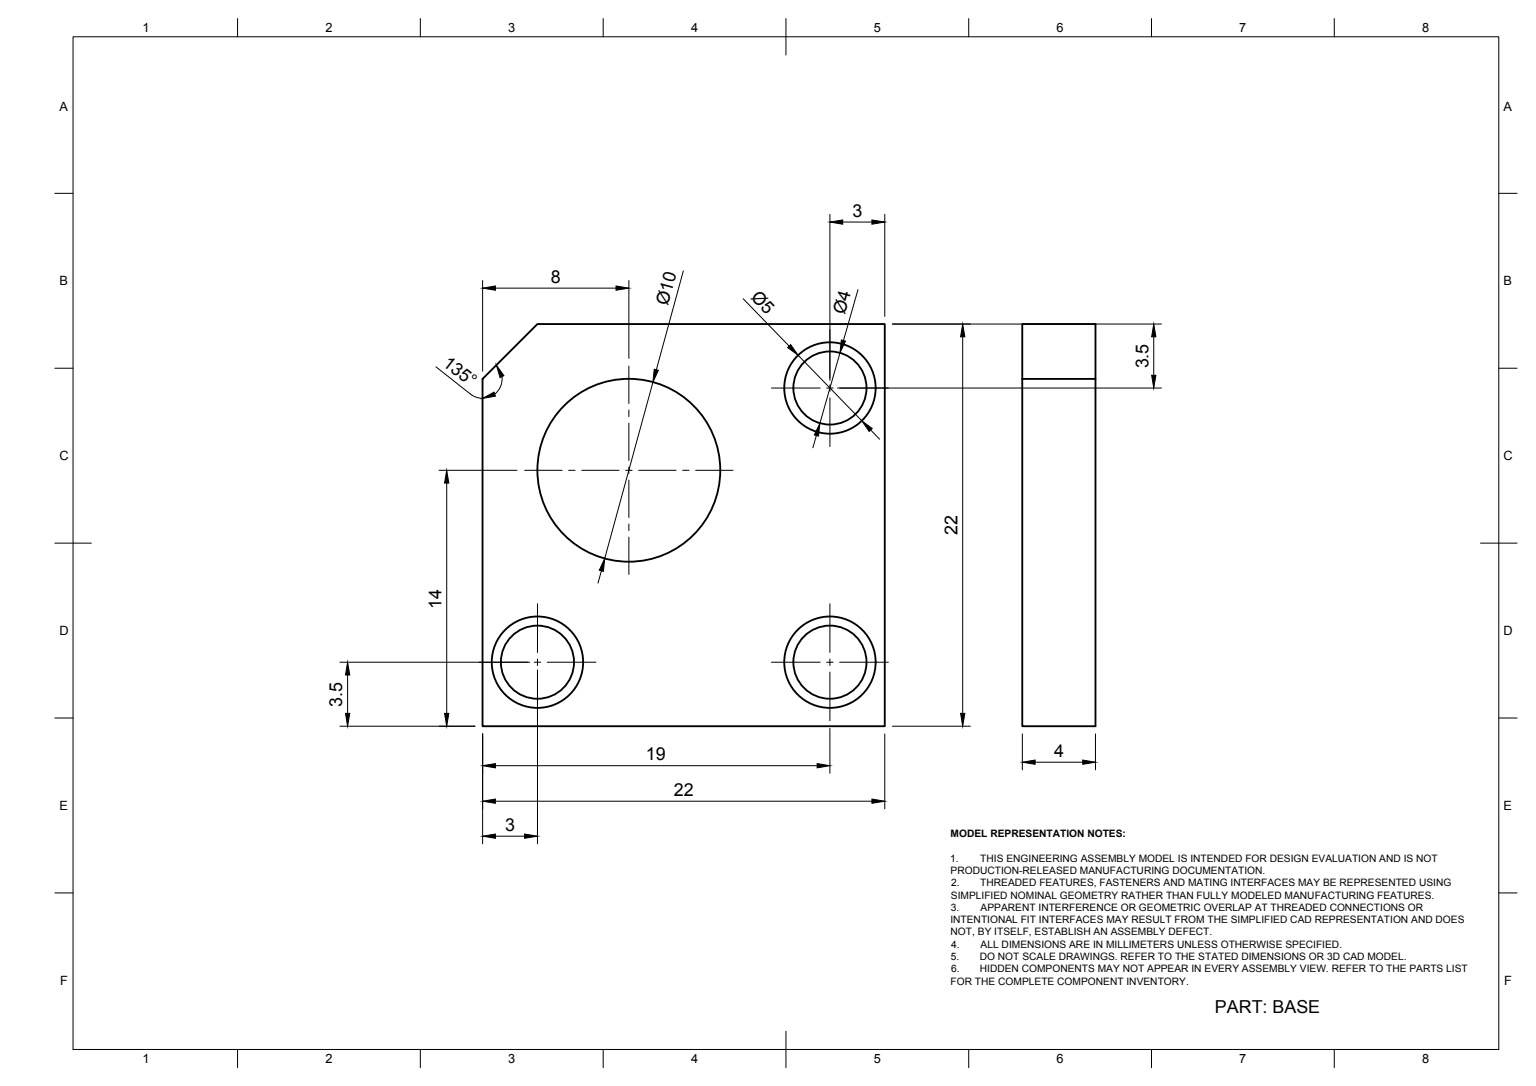
ISO-10303-21;
HEADER;
/* Generated by software containing ST-Developer
 * from STEP Tools, Inc. (www.steptools.com) 
 */

FILE_DESCRIPTION(
/* description */ (''),
/* implementation_level */ '2;1');

FILE_NAME(
/* name */ 'Base.step',
/* time_stamp */ '2026-10-04T23:23:09-07:00',
/* author */ (''),
/* organization */ (''),
/* preprocessor_version */ 'ST-DEVELOPER v20.2',
/* originating_system */ 'Autodesk Translation Framework v15.15.0.0',
/* authorisation */ '');

FILE_SCHEMA (('AUTOMOTIVE_DESIGN { 1 0 10303 214 3 1 1 }'));
ENDSEC;

DATA;
#10=MECHANICAL_DESIGN_GEOMETRIC_PRESENTATION_REPRESENTATION('',(#65),#2676);
#49=SHAPE_REPRESENTATION_RELATIONSHIP('SRR','None',#2708,#57);
#57=ADVANCED_BREP_SHAPE_REPRESENTATION('',(#76),#2668);
#65=STYLED_ITEM('',(#2757),#76);
#76=MANIFOLD_SOLID_BREP('Body1',#1476);
#87=CYLINDRICAL_SURFACE('',#1585,2.);
#88=CYLINDRICAL_SURFACE('',#1589,2.);
#89=CYLINDRICAL_SURFACE('',#1593,2.);
#90=CYLINDRICAL_SURFACE('',#1598,5.);
#109=FACE_BOUND('',#287,.T.);
#110=FACE_BOUND('',#288,.T.);
#111=FACE_BOUND('',#289,.T.);
#112=FACE_BOUND('',#290,.T.);
#113=FACE_BOUND('',#306,.T.);
#135=PLANE('',#1581);
#136=PLANE('',#1595);
#137=PLANE('',#1596);
#138=PLANE('',#1597);
#139=PLANE('',#1600);
#140=PLANE('',#1601);
#141=PLANE('',#1602);
#142=PLANE('',#1603);
#143=PLANE('',#1604);
#144=PLANE('',#1605);
#187=FACE_OUTER_BOUND('',#285,.T.);
#188=FACE_OUTER_BOUND('',#286,.T.);
#189=FACE_OUTER_BOUND('',#291,.T.);
#190=FACE_OUTER_BOUND('',#292,.T.);
#191=FACE_OUTER_BOUND('',#293,.T.);
#192=FACE_OUTER_BOUND('',#294,.T.);
#193=FACE_OUTER_BOUND('',#295,.T.);
#194=FACE_OUTER_BOUND('',#296,.T.);
#195=FACE_OUTER_BOUND('',#297,.T.);
#196=FACE_OUTER_BOUND('',#298,.T.);
#197=FACE_OUTER_BOUND('',#299,.T.);
#198=FACE_OUTER_BOUND('',#300,.T.);
#199=FACE_OUTER_BOUND('',#301,.T.);
#200=FACE_OUTER_BOUND('',#302,.T.);
#201=FACE_OUTER_BOUND('',#303,.T.);
#202=FACE_OUTER_BOUND('',#304,.T.);
#203=FACE_OUTER_BOUND('',#305,.T.);
#285=EDGE_LOOP('',(#998,#999,#1000,#1001));
#286=EDGE_LOOP('',(#1002,#1003,#1004,#1005,#1006));
#287=EDGE_LOOP('',(#1007));
#288=EDGE_LOOP('',(#1008));
#289=EDGE_LOOP('',(#1009));
#290=EDGE_LOOP('',(#1010));
#291=EDGE_LOOP('',(#1011,#1012,#1013,#1014));
#292=EDGE_LOOP('',(#1015,#1016,#1017,#1018));
#293=EDGE_LOOP('',(#1019,#1020,#1021,#1022));
#294=EDGE_LOOP('',(#1023,#1024,#1025,#1026));
#295=EDGE_LOOP('',(#1027,#1028,#1029,#1030));
#296=EDGE_LOOP('',(#1031));
#297=EDGE_LOOP('',(#1032));
#298=EDGE_LOOP('',(#1033));
#299=EDGE_LOOP('',(#1034,#1035,#1036,#1037));
#300=EDGE_LOOP('',(#1038,#1039,#1040,#1041));
#301=EDGE_LOOP('',(#1042,#1043,#1044,#1045));
#302=EDGE_LOOP('',(#1046,#1047,#1048,#1049));
#303=EDGE_LOOP('',(#1050,#1051,#1052,#1053));
#304=EDGE_LOOP('',(#1054,#1055,#1056,#1057));
#305=EDGE_LOOP('',(#1058,#1059,#1060,#1061,#1062));
#306=EDGE_LOOP('',(#1063));
#409=LINE('',#2250,#519);
#410=LINE('',#2255,#520);
#411=LINE('',#2257,#521);
#412=LINE('',#2259,#522);
#413=LINE('',#2261,#523);
#414=LINE('',#2262,#524);
#415=LINE('',#2271,#525);
#416=LINE('',#2276,#526);
#417=LINE('',#2279,#527);
#418=LINE('',#2284,#528);
#419=LINE('',#2287,#529);
#420=LINE('',#2295,#530);
#421=LINE('',#2299,#531);
#422=LINE('',#2300,#532);
#423=LINE('',#2301,#533);
#424=LINE('',#2304,#534);
#425=LINE('',#2305,#535);
#426=LINE('',#2308,#536);
#427=LINE('',#2309,#537);
#428=LINE('',#2312,#538);
#429=LINE('',#2313,#539);
#430=LINE('',#2315,#540);
#519=VECTOR('',#1770,2.25);
#520=VECTOR('',#1775,10.);
#521=VECTOR('',#1776,10.);
#522=VECTOR('',#1777,10.);
#523=VECTOR('',#1778,10.);
#524=VECTOR('',#1779,10.);
#525=VECTOR('',#1788,2.);
#526=VECTOR('',#1795,2.25);
#527=VECTOR('',#1798,2.);
#528=VECTOR('',#1805,2.25);
#529=VECTOR('',#1808,2.);
#530=VECTOR('',#1821,5.);
#531=VECTOR('',#1824,10.);
#532=VECTOR('',#1825,10.);
#533=VECTOR('',#1826,10.);
#534=VECTOR('',#1829,10.);
#535=VECTOR('',#1830,10.);
#536=VECTOR('',#1833,10.);
#537=VECTOR('',#1834,10.);
#538=VECTOR('',#1837,10.);
#539=VECTOR('',#1838,10.);
#540=VECTOR('',#1841,10.);
#629=CIRCLE('',#1579,2.);
#630=CIRCLE('',#1580,2.5);
#631=CIRCLE('',#1582,2.5);
#632=CIRCLE('',#1583,5.);
#633=CIRCLE('',#1584,2.5);
#634=CIRCLE('',#1586,2.);
#635=CIRCLE('',#1588,2.);
#636=CIRCLE('',#1590,2.);
#637=CIRCLE('',#1592,2.);
#638=CIRCLE('',#1594,2.);
#639=CIRCLE('',#1599,5.);
#700=VERTEX_POINT('',#2247);
#701=VERTEX_POINT('',#2249);
#702=VERTEX_POINT('',#2253);
#703=VERTEX_POINT('',#2254);
#704=VERTEX_POINT('',#2256);
#705=VERTEX_POINT('',#2258);
#706=VERTEX_POINT('',#2260);
#707=VERTEX_POINT('',#2263);
#708=VERTEX_POINT('',#2265);
#709=VERTEX_POINT('',#2267);
#710=VERTEX_POINT('',#2270);
#711=VERTEX_POINT('',#2274);
#712=VERTEX_POINT('',#2278);
#713=VERTEX_POINT('',#2282);
#714=VERTEX_POINT('',#2286);
#715=VERTEX_POINT('',#2293);
#716=VERTEX_POINT('',#2297);
#717=VERTEX_POINT('',#2298);
#718=VERTEX_POINT('',#2303);
#719=VERTEX_POINT('',#2307);
#720=VERTEX_POINT('',#2311);
#817=EDGE_CURVE('',#700,#700,#629,.T.);
#818=EDGE_CURVE('',#700,#701,#409,.T.);
#819=EDGE_CURVE('',#701,#701,#630,.T.);
#820=EDGE_CURVE('',#702,#703,#410,.T.);
#821=EDGE_CURVE('',#703,#704,#411,.T.);
#822=EDGE_CURVE('',#704,#705,#412,.T.);
#823=EDGE_CURVE('',#705,#706,#413,.T.);
#824=EDGE_CURVE('',#706,#702,#414,.T.);
#825=EDGE_CURVE('',#707,#707,#631,.T.);
#826=EDGE_CURVE('',#708,#708,#632,.T.);
#827=EDGE_CURVE('',#709,#709,#633,.T.);
#828=EDGE_CURVE('',#700,#710,#415,.T.);
#829=EDGE_CURVE('',#710,#710,#634,.T.);
#830=EDGE_CURVE('',#711,#711,#635,.T.);
#831=EDGE_CURVE('',#711,#707,#416,.T.);
#832=EDGE_CURVE('',#711,#712,#417,.T.);
#833=EDGE_CURVE('',#712,#712,#636,.T.);
#834=EDGE_CURVE('',#713,#713,#637,.T.);
#835=EDGE_CURVE('',#713,#709,#418,.T.);
#836=EDGE_CURVE('',#713,#714,#419,.T.);
#837=EDGE_CURVE('',#714,#714,#638,.T.);
#838=EDGE_CURVE('',#715,#715,#639,.T.);
#839=EDGE_CURVE('',#715,#708,#420,.T.);
#840=EDGE_CURVE('',#716,#717,#421,.T.);
#841=EDGE_CURVE('',#716,#702,#422,.T.);
#842=EDGE_CURVE('',#717,#706,#423,.T.);
#843=EDGE_CURVE('',#718,#717,#424,.T.);
#844=EDGE_CURVE('',#718,#705,#425,.T.);
#845=EDGE_CURVE('',#719,#718,#426,.T.);
#846=EDGE_CURVE('',#719,#704,#427,.T.);
#847=EDGE_CURVE('',#720,#719,#428,.T.);
#848=EDGE_CURVE('',#720,#703,#429,.T.);
#849=EDGE_CURVE('',#716,#720,#430,.T.);
#998=ORIENTED_EDGE('',*,*,#817,.T.);
#999=ORIENTED_EDGE('',*,*,#818,.T.);
#1000=ORIENTED_EDGE('',*,*,#819,.T.);
#1001=ORIENTED_EDGE('',*,*,#818,.F.);
#1002=ORIENTED_EDGE('',*,*,#820,.T.);
#1003=ORIENTED_EDGE('',*,*,#821,.T.);
#1004=ORIENTED_EDGE('',*,*,#822,.T.);
#1005=ORIENTED_EDGE('',*,*,#823,.T.);
#1006=ORIENTED_EDGE('',*,*,#824,.T.);
#1007=ORIENTED_EDGE('',*,*,#825,.F.);
#1008=ORIENTED_EDGE('',*,*,#826,.T.);
#1009=ORIENTED_EDGE('',*,*,#827,.F.);
#1010=ORIENTED_EDGE('',*,*,#819,.F.);
#1011=ORIENTED_EDGE('',*,*,#817,.F.);
#1012=ORIENTED_EDGE('',*,*,#828,.T.);
#1013=ORIENTED_EDGE('',*,*,#829,.T.);
#1014=ORIENTED_EDGE('',*,*,#828,.F.);
#1015=ORIENTED_EDGE('',*,*,#830,.T.);
#1016=ORIENTED_EDGE('',*,*,#831,.T.);
#1017=ORIENTED_EDGE('',*,*,#825,.T.);
#1018=ORIENTED_EDGE('',*,*,#831,.F.);
#1019=ORIENTED_EDGE('',*,*,#830,.F.);
#1020=ORIENTED_EDGE('',*,*,#832,.T.);
#1021=ORIENTED_EDGE('',*,*,#833,.T.);
#1022=ORIENTED_EDGE('',*,*,#832,.F.);
#1023=ORIENTED_EDGE('',*,*,#834,.T.);
#1024=ORIENTED_EDGE('',*,*,#835,.T.);
#1025=ORIENTED_EDGE('',*,*,#827,.T.);
#1026=ORIENTED_EDGE('',*,*,#835,.F.);
#1027=ORIENTED_EDGE('',*,*,#834,.F.);
#1028=ORIENTED_EDGE('',*,*,#836,.T.);
#1029=ORIENTED_EDGE('',*,*,#837,.T.);
#1030=ORIENTED_EDGE('',*,*,#836,.F.);
#1031=ORIENTED_EDGE('',*,*,#837,.F.);
#1032=ORIENTED_EDGE('',*,*,#833,.F.);
#1033=ORIENTED_EDGE('',*,*,#829,.F.);
#1034=ORIENTED_EDGE('',*,*,#838,.T.);
#1035=ORIENTED_EDGE('',*,*,#839,.T.);
#1036=ORIENTED_EDGE('',*,*,#826,.F.);
#1037=ORIENTED_EDGE('',*,*,#839,.F.);
#1038=ORIENTED_EDGE('',*,*,#840,.F.);
#1039=ORIENTED_EDGE('',*,*,#841,.T.);
#1040=ORIENTED_EDGE('',*,*,#824,.F.);
#1041=ORIENTED_EDGE('',*,*,#842,.F.);
#1042=ORIENTED_EDGE('',*,*,#843,.T.);
#1043=ORIENTED_EDGE('',*,*,#842,.T.);
#1044=ORIENTED_EDGE('',*,*,#823,.F.);
#1045=ORIENTED_EDGE('',*,*,#844,.F.);
#1046=ORIENTED_EDGE('',*,*,#845,.T.);
#1047=ORIENTED_EDGE('',*,*,#844,.T.);
#1048=ORIENTED_EDGE('',*,*,#822,.F.);
#1049=ORIENTED_EDGE('',*,*,#846,.F.);
#1050=ORIENTED_EDGE('',*,*,#847,.T.);
#1051=ORIENTED_EDGE('',*,*,#846,.T.);
#1052=ORIENTED_EDGE('',*,*,#821,.F.);
#1053=ORIENTED_EDGE('',*,*,#848,.F.);
#1054=ORIENTED_EDGE('',*,*,#849,.T.);
#1055=ORIENTED_EDGE('',*,*,#848,.T.);
#1056=ORIENTED_EDGE('',*,*,#820,.F.);
#1057=ORIENTED_EDGE('',*,*,#841,.F.);
#1058=ORIENTED_EDGE('',*,*,#849,.F.);
#1059=ORIENTED_EDGE('',*,*,#840,.T.);
#1060=ORIENTED_EDGE('',*,*,#843,.F.);
#1061=ORIENTED_EDGE('',*,*,#845,.F.);
#1062=ORIENTED_EDGE('',*,*,#847,.F.);
#1063=ORIENTED_EDGE('',*,*,#838,.F.);
#1360=CONICAL_SURFACE('',#1578,2.25,0.785398163397449);
#1361=CONICAL_SURFACE('',#1587,2.25,0.785398163397449);
#1362=CONICAL_SURFACE('',#1591,2.25,0.785398163397449);
#1378=ADVANCED_FACE('',(#187),#1360,.F.);
#1379=ADVANCED_FACE('',(#188,#109,#110,#111,#112),#135,.T.);
#1380=ADVANCED_FACE('',(#189),#87,.F.);
#1381=ADVANCED_FACE('',(#190),#1361,.F.);
#1382=ADVANCED_FACE('',(#191),#88,.F.);
#1383=ADVANCED_FACE('',(#192),#1362,.F.);
#1384=ADVANCED_FACE('',(#193),#89,.F.);
#1385=ADVANCED_FACE('',(#194),#136,.T.);
#1386=ADVANCED_FACE('',(#195),#137,.T.);
#1387=ADVANCED_FACE('',(#196),#138,.T.);
#1388=ADVANCED_FACE('',(#197),#90,.F.);
#1389=ADVANCED_FACE('',(#198),#139,.T.);
#1390=ADVANCED_FACE('',(#199),#140,.T.);
#1391=ADVANCED_FACE('',(#200),#141,.T.);
#1392=ADVANCED_FACE('',(#201),#142,.T.);
#1393=ADVANCED_FACE('',(#202),#143,.T.);
#1394=ADVANCED_FACE('',(#203,#113),#144,.F.);
#1476=CLOSED_SHELL('',(#1378,#1379,#1380,#1381,#1382,#1383,#1384,#1385,
#1386,#1387,#1388,#1389,#1390,#1391,#1392,#1393,#1394));
#1577=AXIS2_PLACEMENT_3D('',#2245,#1764,#1765);
#1578=AXIS2_PLACEMENT_3D('',#2246,#1766,#1767);
#1579=AXIS2_PLACEMENT_3D('',#2248,#1768,#1769);
#1580=AXIS2_PLACEMENT_3D('',#2251,#1771,#1772);
#1581=AXIS2_PLACEMENT_3D('',#2252,#1773,#1774);
#1582=AXIS2_PLACEMENT_3D('',#2264,#1780,#1781);
#1583=AXIS2_PLACEMENT_3D('',#2266,#1782,#1783);
#1584=AXIS2_PLACEMENT_3D('',#2268,#1784,#1785);
#1585=AXIS2_PLACEMENT_3D('',#2269,#1786,#1787);
#1586=AXIS2_PLACEMENT_3D('',#2272,#1789,#1790);
#1587=AXIS2_PLACEMENT_3D('',#2273,#1791,#1792);
#1588=AXIS2_PLACEMENT_3D('',#2275,#1793,#1794);
#1589=AXIS2_PLACEMENT_3D('',#2277,#1796,#1797);
#1590=AXIS2_PLACEMENT_3D('',#2280,#1799,#1800);
#1591=AXIS2_PLACEMENT_3D('',#2281,#1801,#1802);
#1592=AXIS2_PLACEMENT_3D('',#2283,#1803,#1804);
#1593=AXIS2_PLACEMENT_3D('',#2285,#1806,#1807);
#1594=AXIS2_PLACEMENT_3D('',#2288,#1809,#1810);
#1595=AXIS2_PLACEMENT_3D('',#2289,#1811,#1812);
#1596=AXIS2_PLACEMENT_3D('',#2290,#1813,#1814);
#1597=AXIS2_PLACEMENT_3D('',#2291,#1815,#1816);
#1598=AXIS2_PLACEMENT_3D('',#2292,#1817,#1818);
#1599=AXIS2_PLACEMENT_3D('',#2294,#1819,#1820);
#1600=AXIS2_PLACEMENT_3D('',#2296,#1822,#1823);
#1601=AXIS2_PLACEMENT_3D('',#2302,#1827,#1828);
#1602=AXIS2_PLACEMENT_3D('',#2306,#1831,#1832);
#1603=AXIS2_PLACEMENT_3D('',#2310,#1835,#1836);
#1604=AXIS2_PLACEMENT_3D('',#2314,#1839,#1840);
#1605=AXIS2_PLACEMENT_3D('',#2316,#1842,#1843);
#1764=DIRECTION('axis',(0.,0.,1.));
#1765=DIRECTION('refdir',(1.,0.,0.));
#1766=DIRECTION('center_axis',(0.,0.,1.));
#1767=DIRECTION('ref_axis',(-1.,0.,0.));
#1768=DIRECTION('center_axis',(0.,0.,-1.));
#1769=DIRECTION('ref_axis',(-1.,0.,0.));
#1770=DIRECTION('',(0.707106781186548,8.65956056235494E-17,0.707106781186547));
#1771=DIRECTION('center_axis',(0.,0.,1.));
#1772=DIRECTION('ref_axis',(-1.,0.,0.));
#1773=DIRECTION('center_axis',(0.,0.,1.));
#1774=DIRECTION('ref_axis',(1.,0.,0.));
#1775=DIRECTION('',(0.,-1.,0.));
#1776=DIRECTION('',(1.,0.,0.));
#1777=DIRECTION('',(0.,1.,0.));
#1778=DIRECTION('',(-1.,0.,0.));
#1779=DIRECTION('',(-0.707106781186547,-0.707106781186547,0.));
#1780=DIRECTION('center_axis',(0.,0.,1.));
#1781=DIRECTION('ref_axis',(-1.,0.,0.));
#1782=DIRECTION('center_axis',(0.,0.,-1.));
#1783=DIRECTION('ref_axis',(1.,0.,0.));
#1784=DIRECTION('center_axis',(0.,0.,1.));
#1785=DIRECTION('ref_axis',(-1.,0.,0.));
#1786=DIRECTION('center_axis',(0.,0.,-1.));
#1787=DIRECTION('ref_axis',(-1.,0.,0.));
#1788=DIRECTION('',(0.,0.,-1.));
#1789=DIRECTION('center_axis',(0.,0.,-1.));
#1790=DIRECTION('ref_axis',(-1.,0.,0.));
#1791=DIRECTION('center_axis',(0.,0.,1.));
#1792=DIRECTION('ref_axis',(-1.,0.,0.));
#1793=DIRECTION('center_axis',(0.,0.,-1.));
#1794=DIRECTION('ref_axis',(-1.,0.,0.));
#1795=DIRECTION('',(0.707106781186548,8.65956056235494E-17,0.707106781186547));
#1796=DIRECTION('center_axis',(0.,0.,-1.));
#1797=DIRECTION('ref_axis',(-1.,0.,0.));
#1798=DIRECTION('',(0.,0.,-1.));
#1799=DIRECTION('center_axis',(0.,0.,-1.));
#1800=DIRECTION('ref_axis',(-1.,0.,0.));
#1801=DIRECTION('center_axis',(0.,0.,1.));
#1802=DIRECTION('ref_axis',(-1.,0.,0.));
#1803=DIRECTION('center_axis',(0.,0.,-1.));
#1804=DIRECTION('ref_axis',(-1.,0.,0.));
#1805=DIRECTION('',(0.707106781186548,8.65956056235494E-17,0.707106781186547));
#1806=DIRECTION('center_axis',(0.,0.,-1.));
#1807=DIRECTION('ref_axis',(-1.,0.,0.));
#1808=DIRECTION('',(0.,0.,-1.));
#1809=DIRECTION('center_axis',(0.,0.,-1.));
#1810=DIRECTION('ref_axis',(-1.,0.,0.));
#1811=DIRECTION('center_axis',(0.,0.,1.));
#1812=DIRECTION('ref_axis',(-1.,0.,0.));
#1813=DIRECTION('center_axis',(0.,0.,1.));
#1814=DIRECTION('ref_axis',(-1.,0.,0.));
#1815=DIRECTION('center_axis',(0.,0.,1.));
#1816=DIRECTION('ref_axis',(-1.,0.,0.));
#1817=DIRECTION('center_axis',(0.,0.,1.));
#1818=DIRECTION('ref_axis',(1.,0.,0.));
#1819=DIRECTION('center_axis',(0.,0.,-1.));
#1820=DIRECTION('ref_axis',(1.,0.,0.));
#1821=DIRECTION('',(0.,0.,1.));
#1822=DIRECTION('center_axis',(-0.707106781186548,0.707106781186548,0.));
#1823=DIRECTION('ref_axis',(-0.707106781186548,-0.707106781186548,0.));
#1824=DIRECTION('',(0.707106781186547,0.707106781186547,0.));
#1825=DIRECTION('',(0.,0.,1.));
#1826=DIRECTION('',(0.,0.,1.));
#1827=DIRECTION('center_axis',(0.,1.,0.));
#1828=DIRECTION('ref_axis',(-1.,0.,0.));
#1829=DIRECTION('',(-1.,0.,0.));
#1830=DIRECTION('',(0.,0.,1.));
#1831=DIRECTION('center_axis',(1.,0.,0.));
#1832=DIRECTION('ref_axis',(0.,1.,0.));
#1833=DIRECTION('',(0.,1.,0.));
#1834=DIRECTION('',(0.,0.,1.));
#1835=DIRECTION('center_axis',(0.,-1.,0.));
#1836=DIRECTION('ref_axis',(1.,0.,0.));
#1837=DIRECTION('',(1.,0.,0.));
#1838=DIRECTION('',(0.,0.,1.));
#1839=DIRECTION('center_axis',(-1.,0.,0.));
#1840=DIRECTION('ref_axis',(0.,-1.,0.));
#1841=DIRECTION('',(0.,-1.,0.));
#1842=DIRECTION('center_axis',(0.,0.,1.));
#1843=DIRECTION('ref_axis',(1.,0.,0.));
#2245=CARTESIAN_POINT('',(0.,0.,0.));
#2246=CARTESIAN_POINT('Origin',(-8.,-7.5,3.75));
#2247=CARTESIAN_POINT('',(-6.,-7.5,3.5));
#2248=CARTESIAN_POINT('Origin',(-8.,-7.5,3.5));
#2249=CARTESIAN_POINT('',(-5.5,-7.5,4.));
#2250=CARTESIAN_POINT('',(-5.75,-7.5,3.75));
#2251=CARTESIAN_POINT('Origin',(-8.,-7.5,4.));
#2252=CARTESIAN_POINT('Origin',(0.,0.,4.));
#2253=CARTESIAN_POINT('',(-11.,8.,4.));
#2254=CARTESIAN_POINT('',(-11.,-11.,4.));
#2255=CARTESIAN_POINT('',(-11.,-5.,4.));
#2256=CARTESIAN_POINT('',(11.,-11.,4.));
#2257=CARTESIAN_POINT('',(-11.,-11.,4.));
#2258=CARTESIAN_POINT('',(11.,11.,4.));
#2259=CARTESIAN_POINT('',(11.,-11.,4.));
#2260=CARTESIAN_POINT('',(-8.,11.,4.));
#2261=CARTESIAN_POINT('',(11.,11.,4.));
#2262=CARTESIAN_POINT('',(-11.,8.,4.));
#2263=CARTESIAN_POINT('',(10.5,-7.5,4.));
#2264=CARTESIAN_POINT('Origin',(8.,-7.5,4.));
#2265=CARTESIAN_POINT('',(-8.,3.,4.));
#2266=CARTESIAN_POINT('Origin',(-3.,3.,4.));
#2267=CARTESIAN_POINT('',(10.5,7.5,4.));
#2268=CARTESIAN_POINT('Origin',(8.,7.5,4.));
#2269=CARTESIAN_POINT('Origin',(-8.,-7.5,4.));
#2270=CARTESIAN_POINT('',(-6.,-7.5,3.));
#2271=CARTESIAN_POINT('',(-6.,-7.5,4.));
#2272=CARTESIAN_POINT('Origin',(-8.,-7.5,3.));
#2273=CARTESIAN_POINT('Origin',(8.,-7.5,3.75));
#2274=CARTESIAN_POINT('',(10.,-7.5,3.5));
#2275=CARTESIAN_POINT('Origin',(8.,-7.5,3.5));
#2276=CARTESIAN_POINT('',(10.25,-7.5,3.75));
#2277=CARTESIAN_POINT('Origin',(8.,-7.5,4.));
#2278=CARTESIAN_POINT('',(10.,-7.5,3.));
#2279=CARTESIAN_POINT('',(10.,-7.5,4.));
#2280=CARTESIAN_POINT('Origin',(8.,-7.5,3.));
#2281=CARTESIAN_POINT('Origin',(8.,7.5,3.75));
#2282=CARTESIAN_POINT('',(10.,7.5,3.5));
#2283=CARTESIAN_POINT('Origin',(8.,7.5,3.5));
#2284=CARTESIAN_POINT('',(10.25,7.5,3.75));
#2285=CARTESIAN_POINT('Origin',(8.,7.5,4.));
#2286=CARTESIAN_POINT('',(10.,7.5,3.));
#2287=CARTESIAN_POINT('',(10.,7.5,4.));
#2288=CARTESIAN_POINT('Origin',(8.,7.5,3.));
#2289=CARTESIAN_POINT('Origin',(8.,7.5,3.));
#2290=CARTESIAN_POINT('Origin',(8.,-7.5,3.));
#2291=CARTESIAN_POINT('Origin',(-8.,-7.5,3.));
#2292=CARTESIAN_POINT('Origin',(-3.,3.,0.));
#2293=CARTESIAN_POINT('',(-8.,3.,0.));
#2294=CARTESIAN_POINT('Origin',(-3.,3.,0.));
#2295=CARTESIAN_POINT('',(-8.,3.,0.));
#2296=CARTESIAN_POINT('Origin',(-8.,11.,0.));
#2297=CARTESIAN_POINT('',(-11.,8.,0.));
#2298=CARTESIAN_POINT('',(-8.,11.,0.));
#2299=CARTESIAN_POINT('',(-11.,8.,0.));
#2300=CARTESIAN_POINT('',(-11.,8.,0.));
#2301=CARTESIAN_POINT('',(-8.,11.,0.));
#2302=CARTESIAN_POINT('Origin',(11.,11.,0.));
#2303=CARTESIAN_POINT('',(11.,11.,0.));
#2304=CARTESIAN_POINT('',(11.,11.,0.));
#2305=CARTESIAN_POINT('',(11.,11.,0.));
#2306=CARTESIAN_POINT('Origin',(11.,-11.,0.));
#2307=CARTESIAN_POINT('',(11.,-11.,0.));
#2308=CARTESIAN_POINT('',(11.,-11.,0.));
#2309=CARTESIAN_POINT('',(11.,-11.,0.));
#2310=CARTESIAN_POINT('Origin',(-11.,-11.,0.));
#2311=CARTESIAN_POINT('',(-11.,-11.,0.));
#2312=CARTESIAN_POINT('',(-11.,-11.,0.));
#2313=CARTESIAN_POINT('',(-11.,-11.,0.));
#2314=CARTESIAN_POINT('Origin',(-11.,8.,0.));
#2315=CARTESIAN_POINT('',(-11.,-5.,0.));
#2316=CARTESIAN_POINT('Origin',(0.,0.,0.));
#2658=UNCERTAINTY_MEASURE_WITH_UNIT(LENGTH_MEASURE(0.01),#2677,
'DISTANCE_ACCURACY_VALUE',
'Maximum model space distance between geometric entities at asserted c
onnectivities');
#2666=UNCERTAINTY_MEASURE_WITH_UNIT(LENGTH_MEASURE(0.01),#2677,
'DISTANCE_ACCURACY_VALUE',
'Maximum model space distance between geometric entities at asserted c
onnectivities');
#2668=(
GEOMETRIC_REPRESENTATION_CONTEXT(3)
GLOBAL_UNCERTAINTY_ASSIGNED_CONTEXT((#2658))
GLOBAL_UNIT_ASSIGNED_CONTEXT((#2677,#2679,#2680))
REPRESENTATION_CONTEXT('','3D')
);
#2676=(
GEOMETRIC_REPRESENTATION_CONTEXT(3)
GLOBAL_UNCERTAINTY_ASSIGNED_CONTEXT((#2666))
GLOBAL_UNIT_ASSIGNED_CONTEXT((#2677,#2679,#2680))
REPRESENTATION_CONTEXT('','3D')
);
#2677=(
LENGTH_UNIT()
NAMED_UNIT(*)
SI_UNIT(.MILLI.,.METRE.)
);
#2679=(
NAMED_UNIT(*)
PLANE_ANGLE_UNIT()
SI_UNIT($,.RADIAN.)
);
#2680=(
NAMED_UNIT(*)
SI_UNIT($,.STERADIAN.)
SOLID_ANGLE_UNIT()
);
#2682=SHAPE_DEFINITION_REPRESENTATION(#2691,#2708);
#2691=PRODUCT_DEFINITION_SHAPE('',$,#2718);
#2708=SHAPE_REPRESENTATION('',(#1577),#2668);
#2716=PRODUCT_DEFINITION_CONTEXT('part definition',#2745,'design');
#2718=PRODUCT_DEFINITION('base','Base',#2727,#2716);
#2727=PRODUCT_DEFINITION_FORMATION('',$,#2748);
#2745=APPLICATION_CONTEXT(
'Core Data for Automotive Mechanical Design Process');
#2746=PRODUCT_CONTEXT('part definition',#2745,'mechanical');
#2748=PRODUCT('base','Base',$,(#2746));
#2757=PRESENTATION_STYLE_ASSIGNMENT((#2759));
#2759=SURFACE_STYLE_USAGE(.BOTH.,#2761);
#2761=SURFACE_SIDE_STYLE('',(#2763));
#2763=SURFACE_STYLE_FILL_AREA(#2765);
#2765=FILL_AREA_STYLE('Opaque(203,203,203)',(#2767));
#2767=FILL_AREA_STYLE_COLOUR('Opaque(203,203,203)',#2769);
#2769=COLOUR_RGB('Opaque(203,203,203)', 0.09019608, 0.27058824, 0.51372549);
ENDSEC;
END-ISO-10303-21;
